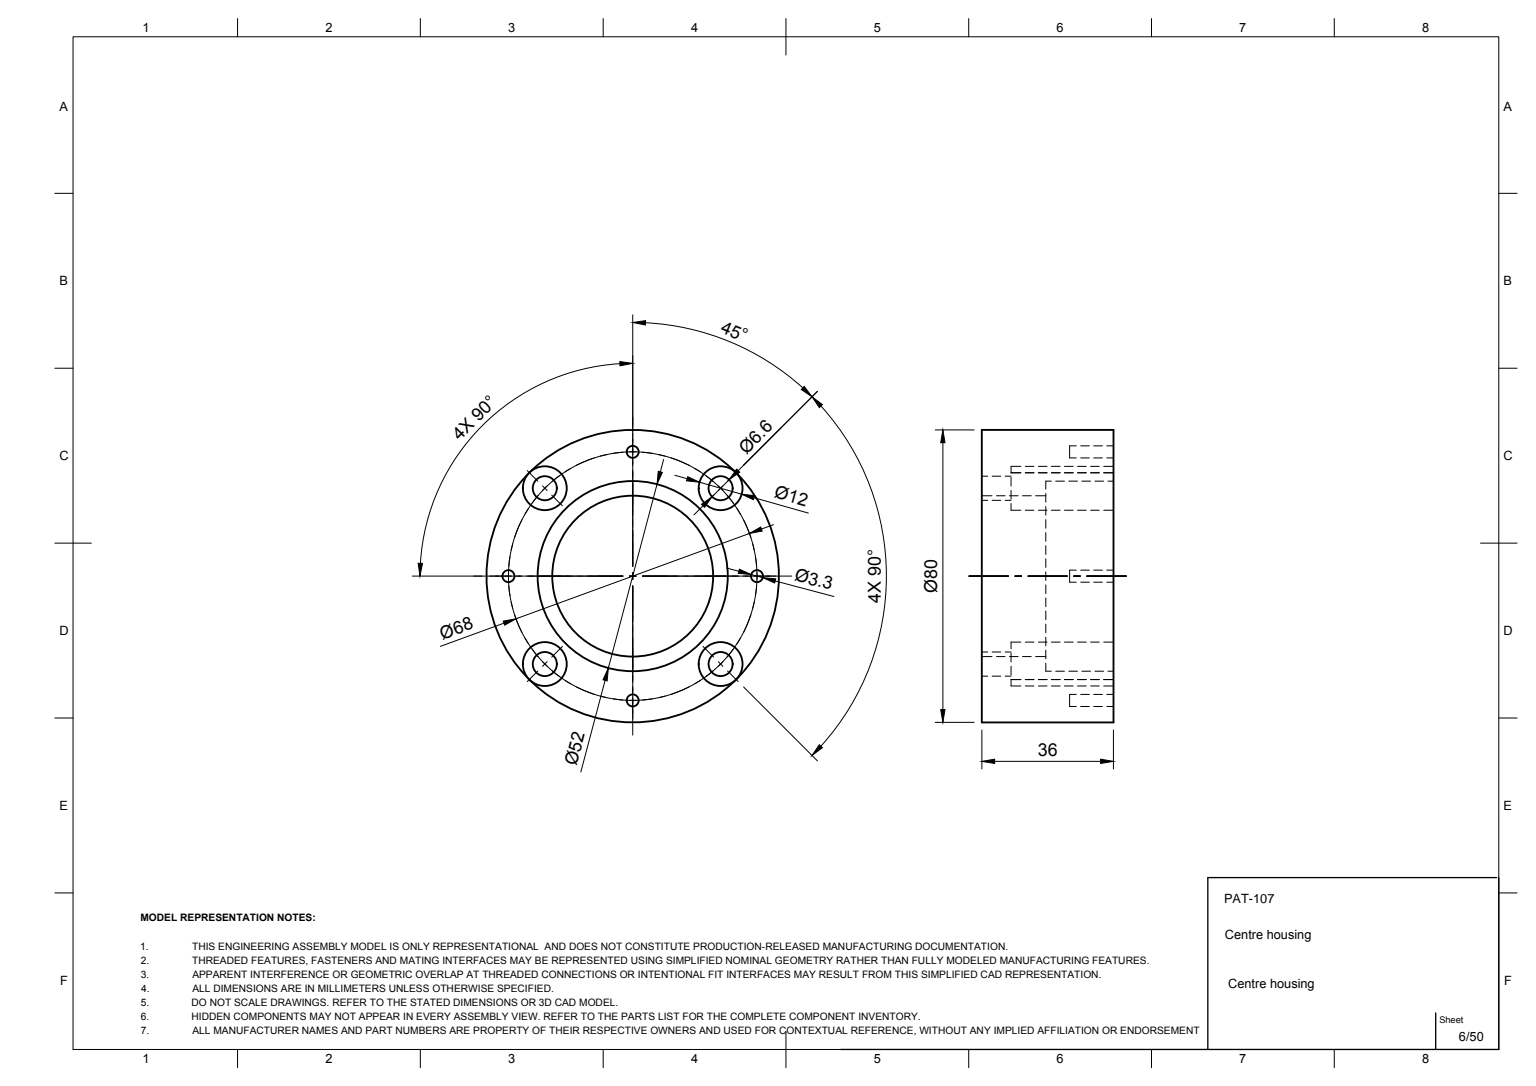
ISO-10303-21;
HEADER;
/* Generated by software containing ST-Developer
 * from STEP Tools, Inc. (www.steptools.com) 
 */

FILE_DESCRIPTION(
/* description */ ('Turntable on roller ring'),
/* implementation_level */ '2;1');

FILE_NAME(
/* name */ 'Centre housing.step',
/* time_stamp */ '2026-10-28T03:23:59-07:00',
/* author */ (''),
/* organization */ (''),
/* preprocessor_version */ 'ST-DEVELOPER v20.2',
/* originating_system */ 'Autodesk Translation Framework v15.17.0.0',
/* authorisation */ '');

FILE_SCHEMA (('AUTOMOTIVE_DESIGN { 1 0 10303 214 3 1 1 }'));
ENDSEC;

DATA;
#10=MECHANICAL_DESIGN_GEOMETRIC_PRESENTATION_REPRESENTATION('',(#618),#16281);
#508=SHAPE_REPRESENTATION_RELATIONSHIP('SRR','None',#16522,#563);
#563=ADVANCED_BREP_SHAPE_REPRESENTATION('',(#690),#16216);
#618=STYLED_ITEM('',(#16911),#690);
#690=MANIFOLD_SOLID_BREP('Body1',#8359);
#797=FACE_BOUND('',#1835,.T.);
#798=FACE_BOUND('',#1838,.T.);
#799=FACE_BOUND('',#1841,.T.);
#800=FACE_BOUND('',#1844,.T.);
#801=FACE_BOUND('',#1846,.T.);
#802=FACE_BOUND('',#1847,.T.);
#803=FACE_BOUND('',#1848,.T.);
#804=FACE_BOUND('',#1849,.T.);
#805=FACE_BOUND('',#1850,.T.);
#806=FACE_BOUND('',#1859,.T.);
#807=FACE_BOUND('',#1861,.T.);
#808=FACE_BOUND('',#1862,.T.);
#809=FACE_BOUND('',#1863,.T.);
#810=FACE_BOUND('',#1864,.T.);
#811=FACE_BOUND('',#1865,.T.);
#996=PLANE('',#9125);
#997=PLANE('',#9129);
#998=PLANE('',#9133);
#999=PLANE('',#9137);
#1000=PLANE('',#9141);
#1001=PLANE('',#9146);
#1002=PLANE('',#9151);
#1003=PLANE('',#9156);
#1004=PLANE('',#9158);
#1005=PLANE('',#9179);
#1006=PLANE('',#9180);
#1276=FACE_OUTER_BOUND('',#1821,.T.);
#1277=FACE_OUTER_BOUND('',#1822,.T.);
#1278=FACE_OUTER_BOUND('',#1823,.T.);
#1279=FACE_OUTER_BOUND('',#1824,.T.);
#1280=FACE_OUTER_BOUND('',#1825,.T.);
#1281=FACE_OUTER_BOUND('',#1826,.T.);
#1282=FACE_OUTER_BOUND('',#1827,.T.);
#1283=FACE_OUTER_BOUND('',#1828,.T.);
#1284=FACE_OUTER_BOUND('',#1829,.T.);
#1285=FACE_OUTER_BOUND('',#1830,.T.);
#1286=FACE_OUTER_BOUND('',#1831,.T.);
#1287=FACE_OUTER_BOUND('',#1832,.T.);
#1288=FACE_OUTER_BOUND('',#1833,.T.);
#1289=FACE_OUTER_BOUND('',#1834,.T.);
#1290=FACE_OUTER_BOUND('',#1836,.T.);
#1291=FACE_OUTER_BOUND('',#1837,.T.);
#1292=FACE_OUTER_BOUND('',#1839,.T.);
#1293=FACE_OUTER_BOUND('',#1840,.T.);
#1294=FACE_OUTER_BOUND('',#1842,.T.);
#1295=FACE_OUTER_BOUND('',#1843,.T.);
#1296=FACE_OUTER_BOUND('',#1845,.T.);
#1297=FACE_OUTER_BOUND('',#1851,.T.);
#1298=FACE_OUTER_BOUND('',#1852,.T.);
#1299=FACE_OUTER_BOUND('',#1853,.T.);
#1300=FACE_OUTER_BOUND('',#1854,.T.);
#1301=FACE_OUTER_BOUND('',#1855,.T.);
#1302=FACE_OUTER_BOUND('',#1856,.T.);
#1303=FACE_OUTER_BOUND('',#1857,.T.);
#1304=FACE_OUTER_BOUND('',#1858,.T.);
#1305=FACE_OUTER_BOUND('',#1860,.T.);
#1821=EDGE_LOOP('',(#5789,#5790,#5791,#5792));
#1822=EDGE_LOOP('',(#5793,#5794,#5795,#5796));
#1823=EDGE_LOOP('',(#5797,#5798,#5799,#5800));
#1824=EDGE_LOOP('',(#5801,#5802,#5803,#5804));
#1825=EDGE_LOOP('',(#5805,#5806,#5807,#5808));
#1826=EDGE_LOOP('',(#5809));
#1827=EDGE_LOOP('',(#5810,#5811,#5812,#5813));
#1828=EDGE_LOOP('',(#5814));
#1829=EDGE_LOOP('',(#5815,#5816,#5817,#5818));
#1830=EDGE_LOOP('',(#5819));
#1831=EDGE_LOOP('',(#5820,#5821,#5822,#5823));
#1832=EDGE_LOOP('',(#5824));
#1833=EDGE_LOOP('',(#5825,#5826,#5827,#5828));
#1834=EDGE_LOOP('',(#5829,#5830));
#1835=EDGE_LOOP('',(#5831));
#1836=EDGE_LOOP('',(#5832,#5833,#5834,#5835));
#1837=EDGE_LOOP('',(#5836,#5837));
#1838=EDGE_LOOP('',(#5838));
#1839=EDGE_LOOP('',(#5839,#5840,#5841,#5842));
#1840=EDGE_LOOP('',(#5843,#5844));
#1841=EDGE_LOOP('',(#5845));
#1842=EDGE_LOOP('',(#5846,#5847,#5848,#5849));
#1843=EDGE_LOOP('',(#5850,#5851));
#1844=EDGE_LOOP('',(#5852));
#1845=EDGE_LOOP('',(#5853,#5854,#5855,#5856,#5857,#5858,#5859,#5860,#5861,
#5862,#5863,#5864));
#1846=EDGE_LOOP('',(#5865));
#1847=EDGE_LOOP('',(#5866));
#1848=EDGE_LOOP('',(#5867));
#1849=EDGE_LOOP('',(#5868));
#1850=EDGE_LOOP('',(#5869));
#1851=EDGE_LOOP('',(#5870,#5871,#5872,#5873));
#1852=EDGE_LOOP('',(#5874,#5875,#5876,#5877));
#1853=EDGE_LOOP('',(#5878,#5879,#5880,#5881));
#1854=EDGE_LOOP('',(#5882,#5883,#5884,#5885));
#1855=EDGE_LOOP('',(#5886,#5887,#5888,#5889));
#1856=EDGE_LOOP('',(#5890,#5891,#5892,#5893));
#1857=EDGE_LOOP('',(#5894,#5895,#5896,#5897,#5898,#5899,#5900,#5901,#5902,
#5903,#5904,#5905,#5906,#5907,#5908));
#1858=EDGE_LOOP('',(#5909));
#1859=EDGE_LOOP('',(#5910));
#1860=EDGE_LOOP('',(#5911));
#1861=EDGE_LOOP('',(#5912));
#1862=EDGE_LOOP('',(#5913));
#1863=EDGE_LOOP('',(#5914));
#1864=EDGE_LOOP('',(#5915));
#1865=EDGE_LOOP('',(#5916));
#2525=LINE('',#13156,#3008);
#2526=LINE('',#13160,#3009);
#2527=LINE('',#13165,#3010);
#2528=LINE('',#13169,#3011);
#2529=LINE('',#13174,#3012);
#2530=LINE('',#13178,#3013);
#2531=LINE('',#13183,#3014);
#2532=LINE('',#13187,#3015);
#2533=LINE('',#13193,#3016);
#2534=LINE('',#13200,#3017);
#2535=LINE('',#13207,#3018);
#2536=LINE('',#13214,#3019);
#2537=LINE('',#13219,#3020);
#2538=LINE('',#13226,#3021);
#2539=LINE('',#13233,#3022);
#2540=LINE('',#13240,#3023);
#2541=LINE('',#13255,#3024);
#2542=LINE('',#13259,#3025);
#2543=LINE('',#13263,#3026);
#2544=LINE('',#13267,#3027);
#2545=LINE('',#13270,#3028);
#2546=LINE('',#13276,#3029);
#2547=LINE('',#13280,#3030);
#3008=VECTOR('',#10374,0.6);
#3009=VECTOR('',#10377,1.);
#3010=VECTOR('',#10382,0.6);
#3011=VECTOR('',#10385,1.);
#3012=VECTOR('',#10390,0.6);
#3013=VECTOR('',#10393,1.);
#3014=VECTOR('',#10398,0.6);
#3015=VECTOR('',#10401,1.);
#3016=VECTOR('',#10408,0.165);
#3017=VECTOR('',#10417,0.165);
#3018=VECTOR('',#10426,0.165);
#3019=VECTOR('',#10435,0.165);
#3020=VECTOR('',#10444,1.);
#3021=VECTOR('',#10455,1.);
#3022=VECTOR('',#10466,1.);
#3023=VECTOR('',#10477,1.);
#3024=VECTOR('',#10500,0.33);
#3025=VECTOR('',#10505,0.33);
#3026=VECTOR('',#10510,0.33);
#3027=VECTOR('',#10515,0.33);
#3028=VECTOR('',#10518,2.6);
#3029=VECTOR('',#10525,2.2);
#3030=VECTOR('',#10530,4.);
#3499=CIRCLE('',#9111,0.6);
#3500=CIRCLE('',#9112,0.6);
#3501=CIRCLE('',#9114,0.6);
#3502=CIRCLE('',#9115,0.6);
#3503=CIRCLE('',#9117,0.6);
#3504=CIRCLE('',#9118,0.6);
#3505=CIRCLE('',#9120,0.6);
#3506=CIRCLE('',#9121,0.6);
#3507=CIRCLE('',#9123,0.165);
#3508=CIRCLE('',#9124,0.165);
#3509=CIRCLE('',#9127,0.165);
#3510=CIRCLE('',#9128,0.165);
#3511=CIRCLE('',#9131,0.165);
#3512=CIRCLE('',#9132,0.165);
#3513=CIRCLE('',#9135,0.165);
#3514=CIRCLE('',#9136,0.165);
#3515=CIRCLE('',#9139,0.6);
#3516=CIRCLE('',#9140,0.6);
#3517=CIRCLE('',#9142,0.33);
#3518=CIRCLE('',#9144,0.6);
#3519=CIRCLE('',#9145,0.6);
#3520=CIRCLE('',#9147,0.33);
#3521=CIRCLE('',#9149,0.6);
#3522=CIRCLE('',#9150,0.6);
#3523=CIRCLE('',#9152,0.33);
#3524=CIRCLE('',#9154,0.6);
#3525=CIRCLE('',#9155,0.6);
#3526=CIRCLE('',#9157,0.33);
#3527=CIRCLE('',#9159,4.);
#3528=CIRCLE('',#9160,4.);
#3529=CIRCLE('',#9161,4.);
#3530=CIRCLE('',#9162,4.);
#3531=CIRCLE('',#9163,2.6);
#3532=CIRCLE('',#9165,0.33);
#3533=CIRCLE('',#9167,0.33);
#3534=CIRCLE('',#9169,0.33);
#3535=CIRCLE('',#9171,0.33);
#3536=CIRCLE('',#9173,2.6);
#3537=CIRCLE('',#9175,2.2);
#3538=CIRCLE('',#9176,2.2);
#3539=CIRCLE('',#9178,4.);
#3997=VERTEX_POINT('',#13154);
#3998=VERTEX_POINT('',#13155);
#3999=VERTEX_POINT('',#13157);
#4000=VERTEX_POINT('',#13159);
#4001=VERTEX_POINT('',#13163);
#4002=VERTEX_POINT('',#13164);
#4003=VERTEX_POINT('',#13166);
#4004=VERTEX_POINT('',#13168);
#4005=VERTEX_POINT('',#13172);
#4006=VERTEX_POINT('',#13173);
#4007=VERTEX_POINT('',#13175);
#4008=VERTEX_POINT('',#13177);
#4009=VERTEX_POINT('',#13181);
#4010=VERTEX_POINT('',#13182);
#4011=VERTEX_POINT('',#13184);
#4012=VERTEX_POINT('',#13186);
#4013=VERTEX_POINT('',#13190);
#4014=VERTEX_POINT('',#13192);
#4015=VERTEX_POINT('',#13197);
#4016=VERTEX_POINT('',#13199);
#4017=VERTEX_POINT('',#13204);
#4018=VERTEX_POINT('',#13206);
#4019=VERTEX_POINT('',#13211);
#4020=VERTEX_POINT('',#13213);
#4021=VERTEX_POINT('',#13222);
#4022=VERTEX_POINT('',#13229);
#4023=VERTEX_POINT('',#13236);
#4024=VERTEX_POINT('',#13243);
#4025=VERTEX_POINT('',#13250);
#4026=VERTEX_POINT('',#13253);
#4027=VERTEX_POINT('',#13257);
#4028=VERTEX_POINT('',#13261);
#4029=VERTEX_POINT('',#13265);
#4030=VERTEX_POINT('',#13269);
#4031=VERTEX_POINT('',#13273);
#4032=VERTEX_POINT('',#13275);
#4033=VERTEX_POINT('',#13279);
#4705=EDGE_CURVE('',#3997,#3998,#2525,.T.);
#4706=EDGE_CURVE('',#3999,#3997,#3499,.T.);
#4707=EDGE_CURVE('',#3999,#4000,#2526,.T.);
#4708=EDGE_CURVE('',#3998,#4000,#3500,.T.);
#4709=EDGE_CURVE('',#4001,#4002,#2527,.T.);
#4710=EDGE_CURVE('',#4003,#4001,#3501,.T.);
#4711=EDGE_CURVE('',#4003,#4004,#2528,.T.);
#4712=EDGE_CURVE('',#4002,#4004,#3502,.T.);
#4713=EDGE_CURVE('',#4005,#4006,#2529,.T.);
#4714=EDGE_CURVE('',#4007,#4005,#3503,.T.);
#4715=EDGE_CURVE('',#4007,#4008,#2530,.T.);
#4716=EDGE_CURVE('',#4006,#4008,#3504,.T.);
#4717=EDGE_CURVE('',#4009,#4010,#2531,.T.);
#4718=EDGE_CURVE('',#4011,#4009,#3505,.T.);
#4719=EDGE_CURVE('',#4011,#4012,#2532,.T.);
#4720=EDGE_CURVE('',#4010,#4012,#3506,.T.);
#4721=EDGE_CURVE('',#4013,#4013,#3507,.T.);
#4722=EDGE_CURVE('',#4013,#4014,#2533,.T.);
#4723=EDGE_CURVE('',#4014,#4014,#3508,.T.);
#4724=EDGE_CURVE('',#4015,#4015,#3509,.T.);
#4725=EDGE_CURVE('',#4015,#4016,#2534,.T.);
#4726=EDGE_CURVE('',#4016,#4016,#3510,.T.);
#4727=EDGE_CURVE('',#4017,#4017,#3511,.T.);
#4728=EDGE_CURVE('',#4017,#4018,#2535,.T.);
#4729=EDGE_CURVE('',#4018,#4018,#3512,.T.);
#4730=EDGE_CURVE('',#4019,#4019,#3513,.T.);
#4731=EDGE_CURVE('',#4019,#4020,#2536,.T.);
#4732=EDGE_CURVE('',#4020,#4020,#3514,.T.);
#4733=EDGE_CURVE('',#4012,#4010,#3515,.T.);
#4734=EDGE_CURVE('',#4011,#4012,#2537,.T.);
#4735=EDGE_CURVE('',#4009,#4011,#3516,.T.);
#4736=EDGE_CURVE('',#4021,#4021,#3517,.T.);
#4737=EDGE_CURVE('',#4008,#4006,#3518,.T.);
#4738=EDGE_CURVE('',#4007,#4008,#2538,.T.);
#4739=EDGE_CURVE('',#4005,#4007,#3519,.T.);
#4740=EDGE_CURVE('',#4022,#4022,#3520,.T.);
#4741=EDGE_CURVE('',#4004,#4002,#3521,.T.);
#4742=EDGE_CURVE('',#4003,#4004,#2539,.T.);
#4743=EDGE_CURVE('',#4001,#4003,#3522,.T.);
#4744=EDGE_CURVE('',#4023,#4023,#3523,.T.);
#4745=EDGE_CURVE('',#4000,#3998,#3524,.T.);
#4746=EDGE_CURVE('',#3999,#4000,#2540,.T.);
#4747=EDGE_CURVE('',#3997,#3999,#3525,.T.);
#4748=EDGE_CURVE('',#4024,#4024,#3526,.T.);
#4749=EDGE_CURVE('',#4008,#4012,#3527,.T.);
#4750=EDGE_CURVE('',#4012,#4000,#3528,.T.);
#4751=EDGE_CURVE('',#4000,#4004,#3529,.T.);
#4752=EDGE_CURVE('',#4004,#4008,#3530,.T.);
#4753=EDGE_CURVE('',#4025,#4025,#3531,.T.);
#4754=EDGE_CURVE('',#4026,#4026,#3532,.T.);
#4755=EDGE_CURVE('',#4026,#4021,#2541,.T.);
#4756=EDGE_CURVE('',#4027,#4027,#3533,.T.);
#4757=EDGE_CURVE('',#4027,#4022,#2542,.T.);
#4758=EDGE_CURVE('',#4028,#4028,#3534,.T.);
#4759=EDGE_CURVE('',#4028,#4023,#2543,.T.);
#4760=EDGE_CURVE('',#4029,#4029,#3535,.T.);
#4761=EDGE_CURVE('',#4029,#4024,#2544,.T.);
#4762=EDGE_CURVE('',#4025,#4030,#2545,.T.);
#4763=EDGE_CURVE('',#4030,#4030,#3536,.T.);
#4764=EDGE_CURVE('',#4031,#4031,#3537,.T.);
#4765=EDGE_CURVE('',#4031,#4032,#2546,.T.);
#4766=EDGE_CURVE('',#4032,#4032,#3538,.T.);
#4767=EDGE_CURVE('',#4007,#4033,#2547,.T.);
#4768=EDGE_CURVE('',#4033,#4033,#3539,.T.);
#5789=ORIENTED_EDGE('',*,*,#4705,.F.);
#5790=ORIENTED_EDGE('',*,*,#4706,.F.);
#5791=ORIENTED_EDGE('',*,*,#4707,.T.);
#5792=ORIENTED_EDGE('',*,*,#4708,.F.);
#5793=ORIENTED_EDGE('',*,*,#4709,.F.);
#5794=ORIENTED_EDGE('',*,*,#4710,.F.);
#5795=ORIENTED_EDGE('',*,*,#4711,.T.);
#5796=ORIENTED_EDGE('',*,*,#4712,.F.);
#5797=ORIENTED_EDGE('',*,*,#4713,.F.);
#5798=ORIENTED_EDGE('',*,*,#4714,.F.);
#5799=ORIENTED_EDGE('',*,*,#4715,.T.);
#5800=ORIENTED_EDGE('',*,*,#4716,.F.);
#5801=ORIENTED_EDGE('',*,*,#4717,.F.);
#5802=ORIENTED_EDGE('',*,*,#4718,.F.);
#5803=ORIENTED_EDGE('',*,*,#4719,.T.);
#5804=ORIENTED_EDGE('',*,*,#4720,.F.);
#5805=ORIENTED_EDGE('',*,*,#4721,.F.);
#5806=ORIENTED_EDGE('',*,*,#4722,.T.);
#5807=ORIENTED_EDGE('',*,*,#4723,.F.);
#5808=ORIENTED_EDGE('',*,*,#4722,.F.);
#5809=ORIENTED_EDGE('',*,*,#4721,.T.);
#5810=ORIENTED_EDGE('',*,*,#4724,.F.);
#5811=ORIENTED_EDGE('',*,*,#4725,.T.);
#5812=ORIENTED_EDGE('',*,*,#4726,.F.);
#5813=ORIENTED_EDGE('',*,*,#4725,.F.);
#5814=ORIENTED_EDGE('',*,*,#4724,.T.);
#5815=ORIENTED_EDGE('',*,*,#4727,.F.);
#5816=ORIENTED_EDGE('',*,*,#4728,.T.);
#5817=ORIENTED_EDGE('',*,*,#4729,.F.);
#5818=ORIENTED_EDGE('',*,*,#4728,.F.);
#5819=ORIENTED_EDGE('',*,*,#4727,.T.);
#5820=ORIENTED_EDGE('',*,*,#4730,.F.);
#5821=ORIENTED_EDGE('',*,*,#4731,.T.);
#5822=ORIENTED_EDGE('',*,*,#4732,.F.);
#5823=ORIENTED_EDGE('',*,*,#4731,.F.);
#5824=ORIENTED_EDGE('',*,*,#4730,.T.);
#5825=ORIENTED_EDGE('',*,*,#4717,.T.);
#5826=ORIENTED_EDGE('',*,*,#4733,.F.);
#5827=ORIENTED_EDGE('',*,*,#4734,.F.);
#5828=ORIENTED_EDGE('',*,*,#4735,.F.);
#5829=ORIENTED_EDGE('',*,*,#4718,.T.);
#5830=ORIENTED_EDGE('',*,*,#4735,.T.);
#5831=ORIENTED_EDGE('',*,*,#4736,.F.);
#5832=ORIENTED_EDGE('',*,*,#4713,.T.);
#5833=ORIENTED_EDGE('',*,*,#4737,.F.);
#5834=ORIENTED_EDGE('',*,*,#4738,.F.);
#5835=ORIENTED_EDGE('',*,*,#4739,.F.);
#5836=ORIENTED_EDGE('',*,*,#4714,.T.);
#5837=ORIENTED_EDGE('',*,*,#4739,.T.);
#5838=ORIENTED_EDGE('',*,*,#4740,.F.);
#5839=ORIENTED_EDGE('',*,*,#4709,.T.);
#5840=ORIENTED_EDGE('',*,*,#4741,.F.);
#5841=ORIENTED_EDGE('',*,*,#4742,.F.);
#5842=ORIENTED_EDGE('',*,*,#4743,.F.);
#5843=ORIENTED_EDGE('',*,*,#4710,.T.);
#5844=ORIENTED_EDGE('',*,*,#4743,.T.);
#5845=ORIENTED_EDGE('',*,*,#4744,.F.);
#5846=ORIENTED_EDGE('',*,*,#4705,.T.);
#5847=ORIENTED_EDGE('',*,*,#4745,.F.);
#5848=ORIENTED_EDGE('',*,*,#4746,.F.);
#5849=ORIENTED_EDGE('',*,*,#4747,.F.);
#5850=ORIENTED_EDGE('',*,*,#4706,.T.);
#5851=ORIENTED_EDGE('',*,*,#4747,.T.);
#5852=ORIENTED_EDGE('',*,*,#4748,.F.);
#5853=ORIENTED_EDGE('',*,*,#4749,.T.);
#5854=ORIENTED_EDGE('',*,*,#4733,.T.);
#5855=ORIENTED_EDGE('',*,*,#4720,.T.);
#5856=ORIENTED_EDGE('',*,*,#4750,.T.);
#5857=ORIENTED_EDGE('',*,*,#4745,.T.);
#5858=ORIENTED_EDGE('',*,*,#4708,.T.);
#5859=ORIENTED_EDGE('',*,*,#4751,.T.);
#5860=ORIENTED_EDGE('',*,*,#4741,.T.);
#5861=ORIENTED_EDGE('',*,*,#4712,.T.);
#5862=ORIENTED_EDGE('',*,*,#4752,.T.);
#5863=ORIENTED_EDGE('',*,*,#4737,.T.);
#5864=ORIENTED_EDGE('',*,*,#4716,.T.);
#5865=ORIENTED_EDGE('',*,*,#4753,.T.);
#5866=ORIENTED_EDGE('',*,*,#4732,.T.);
#5867=ORIENTED_EDGE('',*,*,#4729,.T.);
#5868=ORIENTED_EDGE('',*,*,#4726,.T.);
#5869=ORIENTED_EDGE('',*,*,#4723,.T.);
#5870=ORIENTED_EDGE('',*,*,#4754,.F.);
#5871=ORIENTED_EDGE('',*,*,#4755,.T.);
#5872=ORIENTED_EDGE('',*,*,#4736,.T.);
#5873=ORIENTED_EDGE('',*,*,#4755,.F.);
#5874=ORIENTED_EDGE('',*,*,#4756,.F.);
#5875=ORIENTED_EDGE('',*,*,#4757,.T.);
#5876=ORIENTED_EDGE('',*,*,#4740,.T.);
#5877=ORIENTED_EDGE('',*,*,#4757,.F.);
#5878=ORIENTED_EDGE('',*,*,#4758,.F.);
#5879=ORIENTED_EDGE('',*,*,#4759,.T.);
#5880=ORIENTED_EDGE('',*,*,#4744,.T.);
#5881=ORIENTED_EDGE('',*,*,#4759,.F.);
#5882=ORIENTED_EDGE('',*,*,#4760,.F.);
#5883=ORIENTED_EDGE('',*,*,#4761,.T.);
#5884=ORIENTED_EDGE('',*,*,#4748,.T.);
#5885=ORIENTED_EDGE('',*,*,#4761,.F.);
#5886=ORIENTED_EDGE('',*,*,#4753,.F.);
#5887=ORIENTED_EDGE('',*,*,#4762,.T.);
#5888=ORIENTED_EDGE('',*,*,#4763,.F.);
#5889=ORIENTED_EDGE('',*,*,#4762,.F.);
#5890=ORIENTED_EDGE('',*,*,#4764,.F.);
#5891=ORIENTED_EDGE('',*,*,#4765,.T.);
#5892=ORIENTED_EDGE('',*,*,#4766,.T.);
#5893=ORIENTED_EDGE('',*,*,#4765,.F.);
#5894=ORIENTED_EDGE('',*,*,#4749,.F.);
#5895=ORIENTED_EDGE('',*,*,#4715,.F.);
#5896=ORIENTED_EDGE('',*,*,#4767,.T.);
#5897=ORIENTED_EDGE('',*,*,#4768,.T.);
#5898=ORIENTED_EDGE('',*,*,#4767,.F.);
#5899=ORIENTED_EDGE('',*,*,#4738,.T.);
#5900=ORIENTED_EDGE('',*,*,#4752,.F.);
#5901=ORIENTED_EDGE('',*,*,#4711,.F.);
#5902=ORIENTED_EDGE('',*,*,#4742,.T.);
#5903=ORIENTED_EDGE('',*,*,#4751,.F.);
#5904=ORIENTED_EDGE('',*,*,#4707,.F.);
#5905=ORIENTED_EDGE('',*,*,#4746,.T.);
#5906=ORIENTED_EDGE('',*,*,#4750,.F.);
#5907=ORIENTED_EDGE('',*,*,#4719,.F.);
#5908=ORIENTED_EDGE('',*,*,#4734,.T.);
#5909=ORIENTED_EDGE('',*,*,#4763,.T.);
#5910=ORIENTED_EDGE('',*,*,#4764,.T.);
#5911=ORIENTED_EDGE('',*,*,#4768,.F.);
#5912=ORIENTED_EDGE('',*,*,#4766,.F.);
#5913=ORIENTED_EDGE('',*,*,#4760,.T.);
#5914=ORIENTED_EDGE('',*,*,#4758,.T.);
#5915=ORIENTED_EDGE('',*,*,#4756,.T.);
#5916=ORIENTED_EDGE('',*,*,#4754,.T.);
#7689=CYLINDRICAL_SURFACE('',#9110,0.6);
#7690=CYLINDRICAL_SURFACE('',#9113,0.6);
#7691=CYLINDRICAL_SURFACE('',#9116,0.6);
#7692=CYLINDRICAL_SURFACE('',#9119,0.6);
#7693=CYLINDRICAL_SURFACE('',#9122,0.165);
#7694=CYLINDRICAL_SURFACE('',#9126,0.165);
#7695=CYLINDRICAL_SURFACE('',#9130,0.165);
#7696=CYLINDRICAL_SURFACE('',#9134,0.165);
#7697=CYLINDRICAL_SURFACE('',#9138,0.6);
#7698=CYLINDRICAL_SURFACE('',#9143,0.6);
#7699=CYLINDRICAL_SURFACE('',#9148,0.6);
#7700=CYLINDRICAL_SURFACE('',#9153,0.6);
#7701=CYLINDRICAL_SURFACE('',#9164,0.33);
#7702=CYLINDRICAL_SURFACE('',#9166,0.33);
#7703=CYLINDRICAL_SURFACE('',#9168,0.33);
#7704=CYLINDRICAL_SURFACE('',#9170,0.33);
#7705=CYLINDRICAL_SURFACE('',#9172,2.6);
#7706=CYLINDRICAL_SURFACE('',#9174,2.2);
#7707=CYLINDRICAL_SURFACE('',#9177,4.);
#7879=ADVANCED_FACE('',(#1276),#7689,.F.);
#7880=ADVANCED_FACE('',(#1277),#7690,.F.);
#7881=ADVANCED_FACE('',(#1278),#7691,.F.);
#7882=ADVANCED_FACE('',(#1279),#7692,.F.);
#7883=ADVANCED_FACE('',(#1280),#7693,.F.);
#7884=ADVANCED_FACE('',(#1281),#996,.T.);
#7885=ADVANCED_FACE('',(#1282),#7694,.F.);
#7886=ADVANCED_FACE('',(#1283),#997,.T.);
#7887=ADVANCED_FACE('',(#1284),#7695,.F.);
#7888=ADVANCED_FACE('',(#1285),#998,.T.);
#7889=ADVANCED_FACE('',(#1286),#7696,.F.);
#7890=ADVANCED_FACE('',(#1287),#999,.T.);
#7891=ADVANCED_FACE('',(#1288),#7697,.F.);
#7892=ADVANCED_FACE('',(#1289,#797),#1000,.T.);
#7893=ADVANCED_FACE('',(#1290),#7698,.F.);
#7894=ADVANCED_FACE('',(#1291,#798),#1001,.T.);
#7895=ADVANCED_FACE('',(#1292),#7699,.F.);
#7896=ADVANCED_FACE('',(#1293,#799),#1002,.T.);
#7897=ADVANCED_FACE('',(#1294),#7700,.F.);
#7898=ADVANCED_FACE('',(#1295,#800),#1003,.T.);
#7899=ADVANCED_FACE('',(#1296,#801,#802,#803,#804,#805),#1004,.T.);
#7900=ADVANCED_FACE('',(#1297),#7701,.F.);
#7901=ADVANCED_FACE('',(#1298),#7702,.F.);
#7902=ADVANCED_FACE('',(#1299),#7703,.F.);
#7903=ADVANCED_FACE('',(#1300),#7704,.F.);
#7904=ADVANCED_FACE('',(#1301),#7705,.F.);
#7905=ADVANCED_FACE('',(#1302),#7706,.F.);
#7906=ADVANCED_FACE('',(#1303),#7707,.T.);
#7907=ADVANCED_FACE('',(#1304,#806),#1005,.T.);
#7908=ADVANCED_FACE('',(#1305,#807,#808,#809,#810,#811),#1006,.F.);
#8359=CLOSED_SHELL('',(#7879,#7880,#7881,#7882,#7883,#7884,#7885,#7886,
#7887,#7888,#7889,#7890,#7891,#7892,#7893,#7894,#7895,#7896,#7897,#7898,
#7899,#7900,#7901,#7902,#7903,#7904,#7905,#7906,#7907,#7908));
#9109=AXIS2_PLACEMENT_3D('',#13152,#10370,#10371);
#9110=AXIS2_PLACEMENT_3D('',#13153,#10372,#10373);
#9111=AXIS2_PLACEMENT_3D('',#13158,#10375,#10376);
#9112=AXIS2_PLACEMENT_3D('',#13161,#10378,#10379);
#9113=AXIS2_PLACEMENT_3D('',#13162,#10380,#10381);
#9114=AXIS2_PLACEMENT_3D('',#13167,#10383,#10384);
#9115=AXIS2_PLACEMENT_3D('',#13170,#10386,#10387);
#9116=AXIS2_PLACEMENT_3D('',#13171,#10388,#10389);
#9117=AXIS2_PLACEMENT_3D('',#13176,#10391,#10392);
#9118=AXIS2_PLACEMENT_3D('',#13179,#10394,#10395);
#9119=AXIS2_PLACEMENT_3D('',#13180,#10396,#10397);
#9120=AXIS2_PLACEMENT_3D('',#13185,#10399,#10400);
#9121=AXIS2_PLACEMENT_3D('',#13188,#10402,#10403);
#9122=AXIS2_PLACEMENT_3D('',#13189,#10404,#10405);
#9123=AXIS2_PLACEMENT_3D('',#13191,#10406,#10407);
#9124=AXIS2_PLACEMENT_3D('',#13194,#10409,#10410);
#9125=AXIS2_PLACEMENT_3D('',#13195,#10411,#10412);
#9126=AXIS2_PLACEMENT_3D('',#13196,#10413,#10414);
#9127=AXIS2_PLACEMENT_3D('',#13198,#10415,#10416);
#9128=AXIS2_PLACEMENT_3D('',#13201,#10418,#10419);
#9129=AXIS2_PLACEMENT_3D('',#13202,#10420,#10421);
#9130=AXIS2_PLACEMENT_3D('',#13203,#10422,#10423);
#9131=AXIS2_PLACEMENT_3D('',#13205,#10424,#10425);
#9132=AXIS2_PLACEMENT_3D('',#13208,#10427,#10428);
#9133=AXIS2_PLACEMENT_3D('',#13209,#10429,#10430);
#9134=AXIS2_PLACEMENT_3D('',#13210,#10431,#10432);
#9135=AXIS2_PLACEMENT_3D('',#13212,#10433,#10434);
#9136=AXIS2_PLACEMENT_3D('',#13215,#10436,#10437);
#9137=AXIS2_PLACEMENT_3D('',#13216,#10438,#10439);
#9138=AXIS2_PLACEMENT_3D('',#13217,#10440,#10441);
#9139=AXIS2_PLACEMENT_3D('',#13218,#10442,#10443);
#9140=AXIS2_PLACEMENT_3D('',#13220,#10445,#10446);
#9141=AXIS2_PLACEMENT_3D('',#13221,#10447,#10448);
#9142=AXIS2_PLACEMENT_3D('',#13223,#10449,#10450);
#9143=AXIS2_PLACEMENT_3D('',#13224,#10451,#10452);
#9144=AXIS2_PLACEMENT_3D('',#13225,#10453,#10454);
#9145=AXIS2_PLACEMENT_3D('',#13227,#10456,#10457);
#9146=AXIS2_PLACEMENT_3D('',#13228,#10458,#10459);
#9147=AXIS2_PLACEMENT_3D('',#13230,#10460,#10461);
#9148=AXIS2_PLACEMENT_3D('',#13231,#10462,#10463);
#9149=AXIS2_PLACEMENT_3D('',#13232,#10464,#10465);
#9150=AXIS2_PLACEMENT_3D('',#13234,#10467,#10468);
#9151=AXIS2_PLACEMENT_3D('',#13235,#10469,#10470);
#9152=AXIS2_PLACEMENT_3D('',#13237,#10471,#10472);
#9153=AXIS2_PLACEMENT_3D('',#13238,#10473,#10474);
#9154=AXIS2_PLACEMENT_3D('',#13239,#10475,#10476);
#9155=AXIS2_PLACEMENT_3D('',#13241,#10478,#10479);
#9156=AXIS2_PLACEMENT_3D('',#13242,#10480,#10481);
#9157=AXIS2_PLACEMENT_3D('',#13244,#10482,#10483);
#9158=AXIS2_PLACEMENT_3D('',#13245,#10484,#10485);
#9159=AXIS2_PLACEMENT_3D('',#13246,#10486,#10487);
#9160=AXIS2_PLACEMENT_3D('',#13247,#10488,#10489);
#9161=AXIS2_PLACEMENT_3D('',#13248,#10490,#10491);
#9162=AXIS2_PLACEMENT_3D('',#13249,#10492,#10493);
#9163=AXIS2_PLACEMENT_3D('',#13251,#10494,#10495);
#9164=AXIS2_PLACEMENT_3D('',#13252,#10496,#10497);
#9165=AXIS2_PLACEMENT_3D('',#13254,#10498,#10499);
#9166=AXIS2_PLACEMENT_3D('',#13256,#10501,#10502);
#9167=AXIS2_PLACEMENT_3D('',#13258,#10503,#10504);
#9168=AXIS2_PLACEMENT_3D('',#13260,#10506,#10507);
#9169=AXIS2_PLACEMENT_3D('',#13262,#10508,#10509);
#9170=AXIS2_PLACEMENT_3D('',#13264,#10511,#10512);
#9171=AXIS2_PLACEMENT_3D('',#13266,#10513,#10514);
#9172=AXIS2_PLACEMENT_3D('',#13268,#10516,#10517);
#9173=AXIS2_PLACEMENT_3D('',#13271,#10519,#10520);
#9174=AXIS2_PLACEMENT_3D('',#13272,#10521,#10522);
#9175=AXIS2_PLACEMENT_3D('',#13274,#10523,#10524);
#9176=AXIS2_PLACEMENT_3D('',#13277,#10526,#10527);
#9177=AXIS2_PLACEMENT_3D('',#13278,#10528,#10529);
#9178=AXIS2_PLACEMENT_3D('',#13281,#10531,#10532);
#9179=AXIS2_PLACEMENT_3D('',#13282,#10533,#10534);
#9180=AXIS2_PLACEMENT_3D('',#13283,#10535,#10536);
#10370=DIRECTION('axis',(0.,0.,1.));
#10371=DIRECTION('refdir',(1.,0.,0.));
#10372=DIRECTION('center_axis',(0.,0.,1.));
#10373=DIRECTION('ref_axis',(1.,0.,0.));
#10374=DIRECTION('',(0.,0.,1.));
#10375=DIRECTION('center_axis',(0.,0.,1.));
#10376=DIRECTION('ref_axis',(1.,0.,0.));
#10377=DIRECTION('',(0.,0.,1.));
#10378=DIRECTION('center_axis',(0.,0.,-1.));
#10379=DIRECTION('ref_axis',(1.,0.,0.));
#10380=DIRECTION('center_axis',(0.,0.,1.));
#10381=DIRECTION('ref_axis',(1.,0.,0.));
#10382=DIRECTION('',(0.,0.,1.));
#10383=DIRECTION('center_axis',(0.,0.,1.));
#10384=DIRECTION('ref_axis',(1.,0.,0.));
#10385=DIRECTION('',(0.,0.,1.));
#10386=DIRECTION('center_axis',(0.,0.,-1.));
#10387=DIRECTION('ref_axis',(1.,0.,0.));
#10388=DIRECTION('center_axis',(0.,0.,1.));
#10389=DIRECTION('ref_axis',(1.,0.,0.));
#10390=DIRECTION('',(0.,0.,1.));
#10391=DIRECTION('center_axis',(0.,0.,1.));
#10392=DIRECTION('ref_axis',(1.,0.,0.));
#10393=DIRECTION('',(0.,0.,1.));
#10394=DIRECTION('center_axis',(0.,0.,-1.));
#10395=DIRECTION('ref_axis',(1.,0.,0.));
#10396=DIRECTION('center_axis',(0.,0.,1.));
#10397=DIRECTION('ref_axis',(1.,0.,0.));
#10398=DIRECTION('',(0.,0.,1.));
#10399=DIRECTION('center_axis',(0.,0.,1.));
#10400=DIRECTION('ref_axis',(1.,0.,0.));
#10401=DIRECTION('',(0.,0.,1.));
#10402=DIRECTION('center_axis',(0.,0.,-1.));
#10403=DIRECTION('ref_axis',(1.,0.,0.));
#10404=DIRECTION('center_axis',(0.,0.,1.));
#10405=DIRECTION('ref_axis',(1.,0.,0.));
#10406=DIRECTION('center_axis',(0.,0.,1.));
#10407=DIRECTION('ref_axis',(1.,0.,0.));
#10408=DIRECTION('',(0.,0.,1.));
#10409=DIRECTION('center_axis',(0.,0.,-1.));
#10410=DIRECTION('ref_axis',(1.,0.,0.));
#10411=DIRECTION('center_axis',(0.,0.,1.));
#10412=DIRECTION('ref_axis',(1.,0.,0.));
#10413=DIRECTION('center_axis',(0.,0.,1.));
#10414=DIRECTION('ref_axis',(1.,0.,0.));
#10415=DIRECTION('center_axis',(0.,0.,1.));
#10416=DIRECTION('ref_axis',(1.,0.,0.));
#10417=DIRECTION('',(0.,0.,1.));
#10418=DIRECTION('center_axis',(0.,0.,-1.));
#10419=DIRECTION('ref_axis',(1.,0.,0.));
#10420=DIRECTION('center_axis',(0.,0.,1.));
#10421=DIRECTION('ref_axis',(1.,0.,0.));
#10422=DIRECTION('center_axis',(0.,0.,1.));
#10423=DIRECTION('ref_axis',(1.,0.,0.));
#10424=DIRECTION('center_axis',(0.,0.,1.));
#10425=DIRECTION('ref_axis',(1.,0.,0.));
#10426=DIRECTION('',(0.,0.,1.));
#10427=DIRECTION('center_axis',(0.,0.,-1.));
#10428=DIRECTION('ref_axis',(1.,0.,0.));
#10429=DIRECTION('center_axis',(0.,0.,1.));
#10430=DIRECTION('ref_axis',(1.,0.,0.));
#10431=DIRECTION('center_axis',(0.,0.,1.));
#10432=DIRECTION('ref_axis',(1.,0.,0.));
#10433=DIRECTION('center_axis',(0.,0.,1.));
#10434=DIRECTION('ref_axis',(1.,0.,0.));
#10435=DIRECTION('',(0.,0.,1.));
#10436=DIRECTION('center_axis',(0.,0.,-1.));
#10437=DIRECTION('ref_axis',(1.,0.,0.));
#10438=DIRECTION('center_axis',(0.,0.,1.));
#10439=DIRECTION('ref_axis',(1.,0.,0.));
#10440=DIRECTION('center_axis',(0.,0.,1.));
#10441=DIRECTION('ref_axis',(1.,0.,0.));
#10442=DIRECTION('center_axis',(0.,0.,-1.));
#10443=DIRECTION('ref_axis',(1.,0.,0.));
#10444=DIRECTION('',(0.,0.,1.));
#10445=DIRECTION('center_axis',(0.,0.,1.));
#10446=DIRECTION('ref_axis',(1.,0.,0.));
#10447=DIRECTION('center_axis',(0.,0.,1.));
#10448=DIRECTION('ref_axis',(1.,0.,0.));
#10449=DIRECTION('center_axis',(0.,0.,1.));
#10450=DIRECTION('ref_axis',(1.,0.,0.));
#10451=DIRECTION('center_axis',(0.,0.,1.));
#10452=DIRECTION('ref_axis',(1.,0.,0.));
#10453=DIRECTION('center_axis',(0.,0.,-1.));
#10454=DIRECTION('ref_axis',(1.,0.,0.));
#10455=DIRECTION('',(0.,0.,1.));
#10456=DIRECTION('center_axis',(0.,0.,1.));
#10457=DIRECTION('ref_axis',(1.,0.,0.));
#10458=DIRECTION('center_axis',(0.,0.,1.));
#10459=DIRECTION('ref_axis',(1.,0.,0.));
#10460=DIRECTION('center_axis',(0.,0.,1.));
#10461=DIRECTION('ref_axis',(1.,0.,0.));
#10462=DIRECTION('center_axis',(0.,0.,1.));
#10463=DIRECTION('ref_axis',(1.,0.,0.));
#10464=DIRECTION('center_axis',(0.,0.,-1.));
#10465=DIRECTION('ref_axis',(1.,0.,0.));
#10466=DIRECTION('',(0.,0.,1.));
#10467=DIRECTION('center_axis',(0.,0.,1.));
#10468=DIRECTION('ref_axis',(1.,0.,0.));
#10469=DIRECTION('center_axis',(0.,0.,1.));
#10470=DIRECTION('ref_axis',(1.,0.,0.));
#10471=DIRECTION('center_axis',(0.,0.,1.));
#10472=DIRECTION('ref_axis',(1.,0.,0.));
#10473=DIRECTION('center_axis',(0.,0.,1.));
#10474=DIRECTION('ref_axis',(1.,0.,0.));
#10475=DIRECTION('center_axis',(0.,0.,-1.));
#10476=DIRECTION('ref_axis',(1.,0.,0.));
#10477=DIRECTION('',(0.,0.,1.));
#10478=DIRECTION('center_axis',(0.,0.,1.));
#10479=DIRECTION('ref_axis',(1.,0.,0.));
#10480=DIRECTION('center_axis',(0.,0.,1.));
#10481=DIRECTION('ref_axis',(1.,0.,0.));
#10482=DIRECTION('center_axis',(0.,0.,1.));
#10483=DIRECTION('ref_axis',(1.,0.,0.));
#10484=DIRECTION('center_axis',(0.,0.,1.));
#10485=DIRECTION('ref_axis',(1.,0.,0.));
#10486=DIRECTION('center_axis',(0.,0.,1.));
#10487=DIRECTION('ref_axis',(1.,0.,0.));
#10488=DIRECTION('center_axis',(0.,0.,1.));
#10489=DIRECTION('ref_axis',(1.,0.,0.));
#10490=DIRECTION('center_axis',(0.,0.,1.));
#10491=DIRECTION('ref_axis',(1.,0.,0.));
#10492=DIRECTION('center_axis',(0.,0.,1.));
#10493=DIRECTION('ref_axis',(1.,0.,0.));
#10494=DIRECTION('center_axis',(0.,0.,-1.));
#10495=DIRECTION('ref_axis',(1.,0.,0.));
#10496=DIRECTION('center_axis',(0.,0.,1.));
#10497=DIRECTION('ref_axis',(1.,0.,0.));
#10498=DIRECTION('center_axis',(0.,0.,1.));
#10499=DIRECTION('ref_axis',(1.,0.,0.));
#10500=DIRECTION('',(0.,0.,1.));
#10501=DIRECTION('center_axis',(0.,0.,1.));
#10502=DIRECTION('ref_axis',(1.,0.,0.));
#10503=DIRECTION('center_axis',(0.,0.,1.));
#10504=DIRECTION('ref_axis',(1.,0.,0.));
#10505=DIRECTION('',(0.,0.,1.));
#10506=DIRECTION('center_axis',(0.,0.,1.));
#10507=DIRECTION('ref_axis',(1.,0.,0.));
#10508=DIRECTION('center_axis',(0.,0.,1.));
#10509=DIRECTION('ref_axis',(1.,0.,0.));
#10510=DIRECTION('',(0.,0.,1.));
#10511=DIRECTION('center_axis',(0.,0.,1.));
#10512=DIRECTION('ref_axis',(1.,0.,0.));
#10513=DIRECTION('center_axis',(0.,0.,1.));
#10514=DIRECTION('ref_axis',(1.,0.,0.));
#10515=DIRECTION('',(0.,0.,1.));
#10516=DIRECTION('center_axis',(0.,0.,1.));
#10517=DIRECTION('ref_axis',(1.,0.,0.));
#10518=DIRECTION('',(0.,0.,-1.));
#10519=DIRECTION('center_axis',(0.,0.,1.));
#10520=DIRECTION('ref_axis',(1.,0.,0.));
#10521=DIRECTION('center_axis',(0.,0.,1.));
#10522=DIRECTION('ref_axis',(1.,0.,0.));
#10523=DIRECTION('center_axis',(0.,0.,-1.));
#10524=DIRECTION('ref_axis',(1.,0.,0.));
#10525=DIRECTION('',(0.,0.,-1.));
#10526=DIRECTION('center_axis',(0.,0.,-1.));
#10527=DIRECTION('ref_axis',(1.,0.,0.));
#10528=DIRECTION('center_axis',(0.,0.,1.));
#10529=DIRECTION('ref_axis',(0.707106781186547,-0.707106781186548,0.));
#10530=DIRECTION('',(0.,0.,-1.));
#10531=DIRECTION('center_axis',(0.,0.,1.));
#10532=DIRECTION('ref_axis',(1.,0.,0.));
#10533=DIRECTION('center_axis',(0.,0.,1.));
#10534=DIRECTION('ref_axis',(1.,0.,0.));
#10535=DIRECTION('center_axis',(0.,0.,1.));
#10536=DIRECTION('ref_axis',(1.,0.,0.));
#13152=CARTESIAN_POINT('',(0.,0.,0.));
#13153=CARTESIAN_POINT('Origin',(2.40416305603426,-2.40416305603426,1.8));
#13154=CARTESIAN_POINT('',(1.80416305603426,-2.40416305603426,1.8));
#13155=CARTESIAN_POINT('',(1.80416305603426,-2.40416305603426,4.6));
#13156=CARTESIAN_POINT('',(1.80416305603426,-2.40416305603426,1.8));
#13157=CARTESIAN_POINT('',(2.82842712474619,-2.82842712474619,1.8));
#13158=CARTESIAN_POINT('Origin',(2.40416305603426,-2.40416305603426,1.8));
#13159=CARTESIAN_POINT('',(2.82842712474619,-2.82842712474619,4.6));
#13160=CARTESIAN_POINT('',(2.82842712474619,-2.82842712474619,1.8));
#13161=CARTESIAN_POINT('Origin',(2.40416305603426,-2.40416305603426,4.6));
#13162=CARTESIAN_POINT('Origin',(2.40416305603426,2.40416305603426,1.8));
#13163=CARTESIAN_POINT('',(1.80416305603426,2.40416305603426,1.8));
#13164=CARTESIAN_POINT('',(1.80416305603426,2.40416305603426,4.6));
#13165=CARTESIAN_POINT('',(1.80416305603426,2.40416305603426,1.8));
#13166=CARTESIAN_POINT('',(2.82842712474619,2.82842712474619,1.8));
#13167=CARTESIAN_POINT('Origin',(2.40416305603426,2.40416305603426,1.8));
#13168=CARTESIAN_POINT('',(2.82842712474619,2.82842712474619,4.6));
#13169=CARTESIAN_POINT('',(2.82842712474619,2.82842712474619,1.8));
#13170=CARTESIAN_POINT('Origin',(2.40416305603426,2.40416305603426,4.6));
#13171=CARTESIAN_POINT('Origin',(-2.40416305603426,2.40416305603426,1.8));
#13172=CARTESIAN_POINT('',(-3.00416305603426,2.40416305603426,1.8));
#13173=CARTESIAN_POINT('',(-3.00416305603426,2.40416305603426,4.6));
#13174=CARTESIAN_POINT('',(-3.00416305603426,2.40416305603426,1.8));
#13175=CARTESIAN_POINT('',(-2.82842712474619,2.82842712474619,1.8));
#13176=CARTESIAN_POINT('Origin',(-2.40416305603426,2.40416305603426,1.8));
#13177=CARTESIAN_POINT('',(-2.82842712474619,2.82842712474619,4.6));
#13178=CARTESIAN_POINT('',(-2.82842712474619,2.82842712474619,1.8));
#13179=CARTESIAN_POINT('Origin',(-2.40416305603426,2.40416305603426,4.6));
#13180=CARTESIAN_POINT('Origin',(-2.40416305603426,-2.40416305603426,1.8));
#13181=CARTESIAN_POINT('',(-3.00416305603426,-2.40416305603426,1.8));
#13182=CARTESIAN_POINT('',(-3.00416305603426,-2.40416305603426,4.6));
#13183=CARTESIAN_POINT('',(-3.00416305603426,-2.40416305603426,1.8));
#13184=CARTESIAN_POINT('',(-2.82842712474619,-2.82842712474619,1.8));
#13185=CARTESIAN_POINT('Origin',(-2.40416305603426,-2.40416305603426,1.8));
#13186=CARTESIAN_POINT('',(-2.82842712474619,-2.82842712474619,4.6));
#13187=CARTESIAN_POINT('',(-2.82842712474619,-2.82842712474619,1.8));
#13188=CARTESIAN_POINT('Origin',(-2.40416305603426,-2.40416305603426,4.6));
#13189=CARTESIAN_POINT('Origin',(-3.4,4.163799117101E-16,3.4));
#13190=CARTESIAN_POINT('',(-3.565,3.96173239524169E-16,3.4));
#13191=CARTESIAN_POINT('Origin',(-3.4,4.163799117101E-16,3.4));
#13192=CARTESIAN_POINT('',(-3.565,4.36586583896031E-16,4.6));
#13193=CARTESIAN_POINT('',(-3.565,3.96173239524169E-16,3.4));
#13194=CARTESIAN_POINT('Origin',(-3.4,4.163799117101E-16,4.6));
#13195=CARTESIAN_POINT('Origin',(-3.4,4.16333634234434E-16,3.4));
#13196=CARTESIAN_POINT('Origin',(2.0818995585505E-16,3.4,3.4));
#13197=CARTESIAN_POINT('',(-0.165,3.4,3.4));
#13198=CARTESIAN_POINT('Origin',(2.0818995585505E-16,3.4,3.4));
#13199=CARTESIAN_POINT('',(-0.165,3.4,4.6));
#13200=CARTESIAN_POINT('',(-0.165,3.4,3.4));
#13201=CARTESIAN_POINT('Origin',(2.0818995585505E-16,3.4,4.6));
#13202=CARTESIAN_POINT('Origin',(2.22044604925031E-16,3.4,3.4));
#13203=CARTESIAN_POINT('Origin',(3.4,0.,3.4));
#13204=CARTESIAN_POINT('',(3.235,-2.02066721859313E-17,3.4));
#13205=CARTESIAN_POINT('Origin',(3.4,0.,3.4));
#13206=CARTESIAN_POINT('',(3.235,2.02066721859313E-17,4.6));
#13207=CARTESIAN_POINT('',(3.235,-2.02066721859313E-17,3.4));
#13208=CARTESIAN_POINT('Origin',(3.4,0.,4.6));
#13209=CARTESIAN_POINT('Origin',(3.4,0.,3.4));
#13210=CARTESIAN_POINT('Origin',(-6.2456986756515E-16,-3.4,3.4));
#13211=CARTESIAN_POINT('',(-0.165000000000001,-3.4,3.4));
#13212=CARTESIAN_POINT('Origin',(-6.2456986756515E-16,-3.4,3.4));
#13213=CARTESIAN_POINT('',(-0.165000000000001,-3.4,4.6));
#13214=CARTESIAN_POINT('',(-0.165000000000001,-3.4,3.4));
#13215=CARTESIAN_POINT('Origin',(-6.2456986756515E-16,-3.4,4.6));
#13216=CARTESIAN_POINT('Origin',(-6.38378239159465E-16,-3.4,3.4));
#13217=CARTESIAN_POINT('Origin',(-2.40416305603426,-2.40416305603426,1.8));
#13218=CARTESIAN_POINT('Origin',(-2.40416305603426,-2.40416305603426,4.6));
#13219=CARTESIAN_POINT('',(-2.82842712474619,-2.82842712474619,1.8));
#13220=CARTESIAN_POINT('Origin',(-2.40416305603426,-2.40416305603426,1.8));
#13221=CARTESIAN_POINT('Origin',(-2.40416305603426,-2.40416305603426,1.8));
#13222=CARTESIAN_POINT('',(-2.73416305603426,-2.40416305603426,1.8));
#13223=CARTESIAN_POINT('Origin',(-2.40416305603426,-2.40416305603426,1.8));
#13224=CARTESIAN_POINT('Origin',(-2.40416305603426,2.40416305603426,1.8));
#13225=CARTESIAN_POINT('Origin',(-2.40416305603426,2.40416305603426,4.6));
#13226=CARTESIAN_POINT('',(-2.82842712474619,2.82842712474619,1.8));
#13227=CARTESIAN_POINT('Origin',(-2.40416305603426,2.40416305603426,1.8));
#13228=CARTESIAN_POINT('Origin',(-2.40416305603426,2.40416305603426,1.8));
#13229=CARTESIAN_POINT('',(-2.73416305603426,2.40416305603426,1.8));
#13230=CARTESIAN_POINT('Origin',(-2.40416305603426,2.40416305603426,1.8));
#13231=CARTESIAN_POINT('Origin',(2.40416305603426,2.40416305603426,1.8));
#13232=CARTESIAN_POINT('Origin',(2.40416305603426,2.40416305603426,4.6));
#13233=CARTESIAN_POINT('',(2.82842712474619,2.82842712474619,1.8));
#13234=CARTESIAN_POINT('Origin',(2.40416305603426,2.40416305603426,1.8));
#13235=CARTESIAN_POINT('Origin',(2.40416305603426,2.40416305603426,1.8));
#13236=CARTESIAN_POINT('',(2.07416305603426,2.40416305603426,1.8));
#13237=CARTESIAN_POINT('Origin',(2.40416305603426,2.40416305603426,1.8));
#13238=CARTESIAN_POINT('Origin',(2.40416305603426,-2.40416305603426,1.8));
#13239=CARTESIAN_POINT('Origin',(2.40416305603426,-2.40416305603426,4.6));
#13240=CARTESIAN_POINT('',(2.82842712474619,-2.82842712474619,1.8));
#13241=CARTESIAN_POINT('Origin',(2.40416305603426,-2.40416305603426,1.8));
#13242=CARTESIAN_POINT('Origin',(2.40416305603426,-2.40416305603426,1.8));
#13243=CARTESIAN_POINT('',(2.07416305603426,-2.40416305603426,1.8));
#13244=CARTESIAN_POINT('Origin',(2.40416305603426,-2.40416305603426,1.8));
#13245=CARTESIAN_POINT('Origin',(0.,0.,4.6));
#13246=CARTESIAN_POINT('Origin',(0.,0.,4.6));
#13247=CARTESIAN_POINT('Origin',(0.,0.,4.6));
#13248=CARTESIAN_POINT('Origin',(0.,0.,4.6));
#13249=CARTESIAN_POINT('Origin',(0.,0.,4.6));
#13250=CARTESIAN_POINT('',(-2.6,-3.18408167778312E-16,4.6));
#13251=CARTESIAN_POINT('Origin',(0.,0.,4.6));
#13252=CARTESIAN_POINT('Origin',(-2.40416305603426,-2.40416305603426,0.9));
#13253=CARTESIAN_POINT('',(-2.73416305603426,-2.40416305603426,1.));
#13254=CARTESIAN_POINT('Origin',(-2.40416305603426,-2.40416305603426,1.));
#13255=CARTESIAN_POINT('',(-2.73416305603426,-2.40416305603426,0.9));
#13256=CARTESIAN_POINT('Origin',(-2.40416305603426,2.40416305603426,0.9));
#13257=CARTESIAN_POINT('',(-2.73416305603426,2.40416305603426,1.));
#13258=CARTESIAN_POINT('Origin',(-2.40416305603426,2.40416305603426,1.));
#13259=CARTESIAN_POINT('',(-2.73416305603426,2.40416305603426,0.9));
#13260=CARTESIAN_POINT('Origin',(2.40416305603426,2.40416305603426,0.9));
#13261=CARTESIAN_POINT('',(2.07416305603426,2.40416305603426,1.));
#13262=CARTESIAN_POINT('Origin',(2.40416305603426,2.40416305603426,1.));
#13263=CARTESIAN_POINT('',(2.07416305603426,2.40416305603426,0.9));
#13264=CARTESIAN_POINT('Origin',(2.40416305603426,-2.40416305603426,0.9));
#13265=CARTESIAN_POINT('',(2.07416305603426,-2.40416305603426,1.));
#13266=CARTESIAN_POINT('Origin',(2.40416305603426,-2.40416305603426,1.));
#13267=CARTESIAN_POINT('',(2.07416305603426,-2.40416305603426,0.9));
#13268=CARTESIAN_POINT('Origin',(0.,0.,2.75));
#13269=CARTESIAN_POINT('',(-2.6,-3.18408167778312E-16,2.75));
#13270=CARTESIAN_POINT('',(-2.6,-3.18408167778312E-16,2.75));
#13271=CARTESIAN_POINT('Origin',(0.,0.,2.75));
#13272=CARTESIAN_POINT('Origin',(0.,0.,1.));
#13273=CARTESIAN_POINT('',(-2.2,-2.69422295812418E-16,2.75));
#13274=CARTESIAN_POINT('Origin',(0.,0.,2.75));
#13275=CARTESIAN_POINT('',(-2.2,-2.69422295812418E-16,1.));
#13276=CARTESIAN_POINT('',(-2.2,-2.69422295812418E-16,1.));
#13277=CARTESIAN_POINT('Origin',(0.,0.,1.));
#13278=CARTESIAN_POINT('Origin',(0.,0.,1.));
#13279=CARTESIAN_POINT('',(-2.82842712474619,2.82842712474619,1.));
#13280=CARTESIAN_POINT('',(-2.82842712474619,2.82842712474619,1.));
#13281=CARTESIAN_POINT('Origin',(0.,0.,1.));
#13282=CARTESIAN_POINT('Origin',(0.,0.,2.75));
#13283=CARTESIAN_POINT('Origin',(0.,0.,1.));
#16147=UNCERTAINTY_MEASURE_WITH_UNIT(LENGTH_MEASURE(0.001),#16282,
'DISTANCE_ACCURACY_VALUE',
'Maximum model space distance between geometric entities at asserted c
onnectivities');
#16212=UNCERTAINTY_MEASURE_WITH_UNIT(LENGTH_MEASURE(0.001),#16282,
'DISTANCE_ACCURACY_VALUE',
'Maximum model space distance between geometric entities at asserted c
onnectivities');
#16216=(
GEOMETRIC_REPRESENTATION_CONTEXT(3)
GLOBAL_UNCERTAINTY_ASSIGNED_CONTEXT((#16147))
GLOBAL_UNIT_ASSIGNED_CONTEXT((#16282,#16284,#16285))
REPRESENTATION_CONTEXT('','3D')
);
#16281=(
GEOMETRIC_REPRESENTATION_CONTEXT(3)
GLOBAL_UNCERTAINTY_ASSIGNED_CONTEXT((#16212))
GLOBAL_UNIT_ASSIGNED_CONTEXT((#16282,#16284,#16285))
REPRESENTATION_CONTEXT('','3D')
);
#16282=(
LENGTH_UNIT()
NAMED_UNIT(*)
SI_UNIT(.CENTI.,.METRE.)
);
#16284=(
NAMED_UNIT(*)
PLANE_ANGLE_UNIT()
SI_UNIT($,.RADIAN.)
);
#16285=(
NAMED_UNIT(*)
SI_UNIT($,.STERADIAN.)
SOLID_ANGLE_UNIT()
);
#16289=SHAPE_DEFINITION_REPRESENTATION(#16357,#16522);
#16357=PRODUCT_DEFINITION_SHAPE('',$,#16591);
#16522=SHAPE_REPRESENTATION('',(#9109),#16216);
#16587=PRODUCT_DEFINITION_CONTEXT('part definition',#16793,'design');
#16591=PRODUCT_DEFINITION('Centre housing','Centre housing',#16659,#16587);
#16659=PRODUCT_DEFINITION_FORMATION('',$,#16798);
#16793=APPLICATION_CONTEXT(
'Core Data for Automotive Mechanical Design Process');
#16794=PRODUCT_CONTEXT('part definition',#16793,'mechanical');
#16798=PRODUCT('Centre housing','Centre housing','Centre housing',(#16794));
#16905=COLOUR_RGB('Dark Blue',0.08,0.2,0.34);
#16906=FILL_AREA_STYLE_COLOUR('',#16905);
#16907=FILL_AREA_STYLE('',(#16906));
#16908=SURFACE_STYLE_FILL_AREA(#16907);
#16909=SURFACE_SIDE_STYLE('',(#16908));
#16910=SURFACE_STYLE_USAGE(.BOTH.,#16909);
#16911=PRESENTATION_STYLE_ASSIGNMENT((#16910));
ENDSEC;
END-ISO-10303-21;
